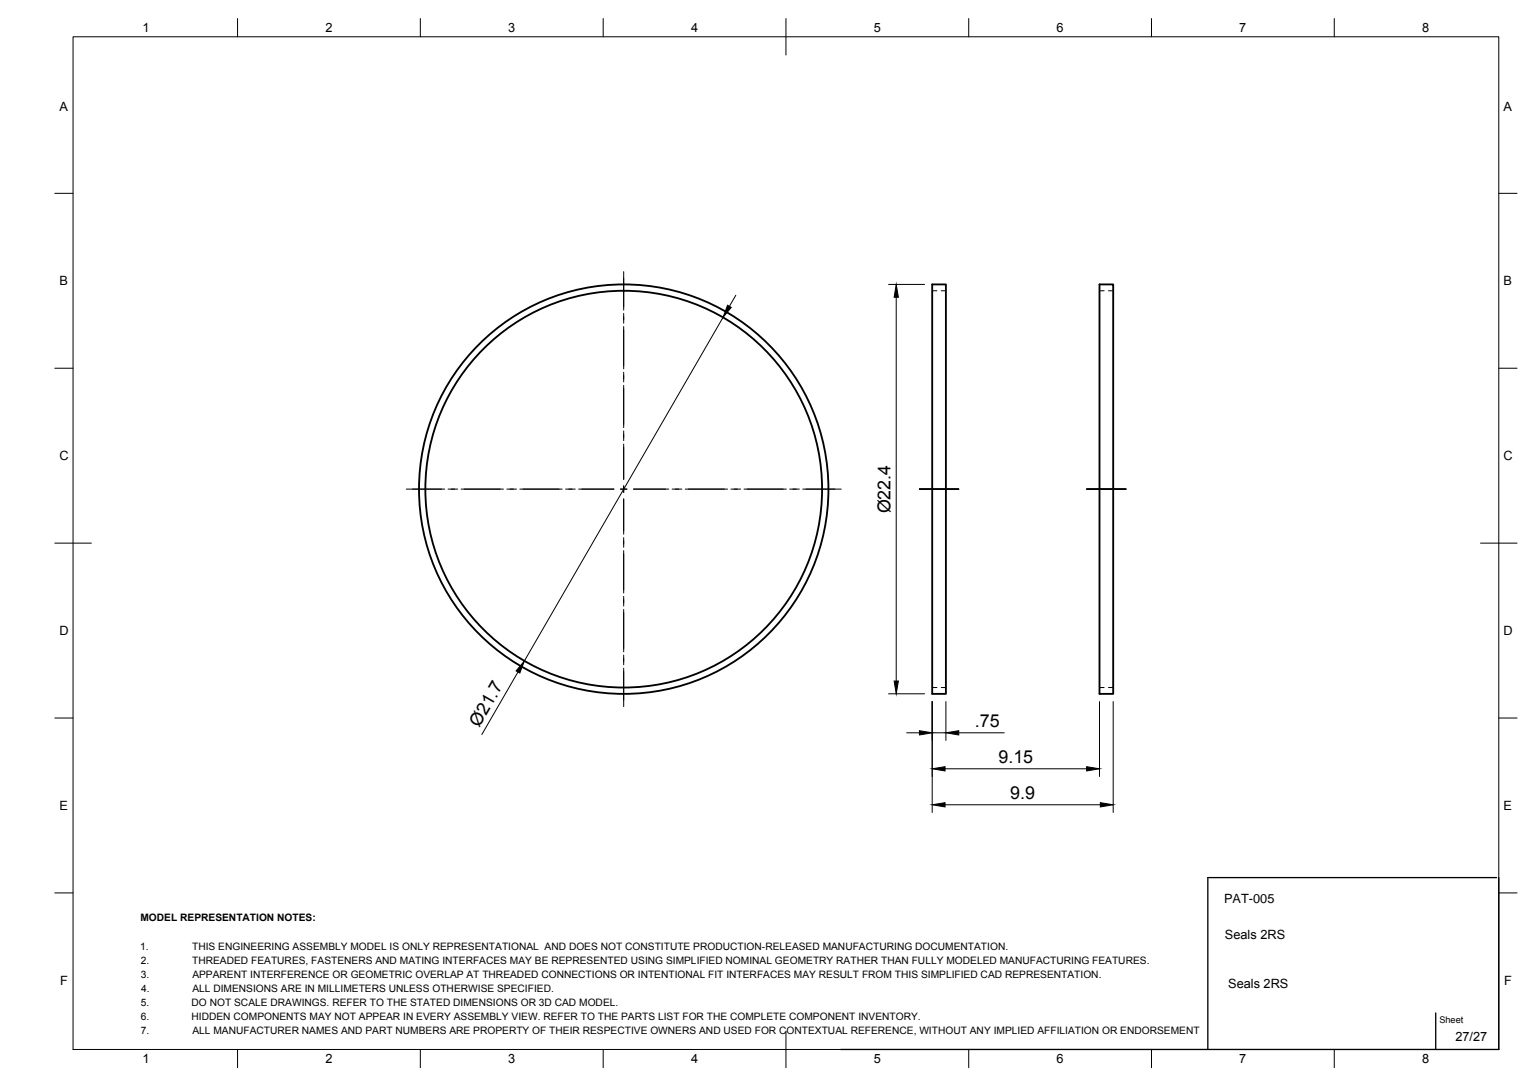
ISO-10303-21;
HEADER;
/* Generated by software containing ST-Developer
 * from STEP Tools, Inc. (www.steptools.com) 
 */

FILE_DESCRIPTION(
/* description */ ('Ball-race swivel caster'),
/* implementation_level */ '2;1');

FILE_NAME(
/* name */ 'Seals 2RS.step',
/* time_stamp */ '2026-10-29T16:15:51-07:00',
/* author */ (''),
/* organization */ (''),
/* preprocessor_version */ 'ST-DEVELOPER v20.2',
/* originating_system */ 'Autodesk Translation Framework v15.17.0.0',
/* authorisation */ '');

FILE_SCHEMA (('AUTOMOTIVE_DESIGN { 1 0 10303 214 3 1 1 }'));
ENDSEC;

DATA;
#10=MECHANICAL_DESIGN_GEOMETRIC_PRESENTATION_REPRESENTATION('',(#331,#332),#7816);
#276=SHAPE_REPRESENTATION_RELATIONSHIP('SRR','None',#7925,#296);
#296=ADVANCED_BREP_SHAPE_REPRESENTATION('',(#366,#367),#7814);
#331=STYLED_ITEM('',(#8097),#366);
#332=STYLED_ITEM('',(#8097),#367);
#366=MANIFOLD_SOLID_BREP('Body1',#3738);
#367=MANIFOLD_SOLID_BREP('Body2',#3739);
#432=FACE_BOUND('',#994,.T.);
#433=FACE_BOUND('',#997,.T.);
#434=FACE_BOUND('',#1000,.T.);
#435=FACE_BOUND('',#1003,.T.);
#518=PLANE('',#4451);
#519=PLANE('',#4456);
#520=PLANE('',#4459);
#521=PLANE('',#4464);
#721=FACE_OUTER_BOUND('',#993,.T.);
#722=FACE_OUTER_BOUND('',#995,.T.);
#723=FACE_OUTER_BOUND('',#996,.T.);
#724=FACE_OUTER_BOUND('',#998,.T.);
#725=FACE_OUTER_BOUND('',#999,.T.);
#726=FACE_OUTER_BOUND('',#1001,.T.);
#727=FACE_OUTER_BOUND('',#1002,.T.);
#728=FACE_OUTER_BOUND('',#1004,.T.);
#993=EDGE_LOOP('',(#3391));
#994=EDGE_LOOP('',(#3392));
#995=EDGE_LOOP('',(#3393,#3394,#3395,#3396));
#996=EDGE_LOOP('',(#3397));
#997=EDGE_LOOP('',(#3398));
#998=EDGE_LOOP('',(#3399,#3400,#3401,#3402));
#999=EDGE_LOOP('',(#3403));
#1000=EDGE_LOOP('',(#3404));
#1001=EDGE_LOOP('',(#3405,#3406,#3407,#3408));
#1002=EDGE_LOOP('',(#3409));
#1003=EDGE_LOOP('',(#3410));
#1004=EDGE_LOOP('',(#3411,#3412,#3413,#3414));
#1160=LINE('',#7715,#1315);
#1161=LINE('',#7720,#1316);
#1162=LINE('',#7729,#1317);
#1163=LINE('',#7734,#1318);
#1315=VECTOR('',#5626,1.119765);
#1316=VECTOR('',#5633,1.085235);
#1317=VECTOR('',#5644,1.119765);
#1318=VECTOR('',#5651,1.085235);
#1573=CIRCLE('',#4452,1.119765);
#1574=CIRCLE('',#4453,1.085235);
#1575=CIRCLE('',#4455,1.119765);
#1576=CIRCLE('',#4457,1.085235);
#1577=CIRCLE('',#4460,1.119765);
#1578=CIRCLE('',#4461,1.085235);
#1579=CIRCLE('',#4463,1.119765);
#1580=CIRCLE('',#4465,1.085235);
#1924=VERTEX_POINT('',#7708);
#1925=VERTEX_POINT('',#7710);
#1926=VERTEX_POINT('',#7713);
#1927=VERTEX_POINT('',#7717);
#1928=VERTEX_POINT('',#7722);
#1929=VERTEX_POINT('',#7724);
#1930=VERTEX_POINT('',#7727);
#1931=VERTEX_POINT('',#7731);
#2415=EDGE_CURVE('',#1924,#1924,#1573,.T.);
#2416=EDGE_CURVE('',#1925,#1925,#1574,.T.);
#2417=EDGE_CURVE('',#1926,#1926,#1575,.T.);
#2418=EDGE_CURVE('',#1926,#1924,#1160,.T.);
#2419=EDGE_CURVE('',#1927,#1927,#1576,.T.);
#2420=EDGE_CURVE('',#1927,#1925,#1161,.T.);
#2421=EDGE_CURVE('',#1928,#1928,#1577,.T.);
#2422=EDGE_CURVE('',#1929,#1929,#1578,.T.);
#2423=EDGE_CURVE('',#1930,#1930,#1579,.T.);
#2424=EDGE_CURVE('',#1930,#1928,#1162,.T.);
#2425=EDGE_CURVE('',#1931,#1931,#1580,.T.);
#2426=EDGE_CURVE('',#1931,#1929,#1163,.T.);
#3391=ORIENTED_EDGE('',*,*,#2415,.F.);
#3392=ORIENTED_EDGE('',*,*,#2416,.T.);
#3393=ORIENTED_EDGE('',*,*,#2417,.F.);
#3394=ORIENTED_EDGE('',*,*,#2418,.T.);
#3395=ORIENTED_EDGE('',*,*,#2415,.T.);
#3396=ORIENTED_EDGE('',*,*,#2418,.F.);
#3397=ORIENTED_EDGE('',*,*,#2417,.T.);
#3398=ORIENTED_EDGE('',*,*,#2419,.F.);
#3399=ORIENTED_EDGE('',*,*,#2419,.T.);
#3400=ORIENTED_EDGE('',*,*,#2420,.T.);
#3401=ORIENTED_EDGE('',*,*,#2416,.F.);
#3402=ORIENTED_EDGE('',*,*,#2420,.F.);
#3403=ORIENTED_EDGE('',*,*,#2421,.F.);
#3404=ORIENTED_EDGE('',*,*,#2422,.T.);
#3405=ORIENTED_EDGE('',*,*,#2423,.F.);
#3406=ORIENTED_EDGE('',*,*,#2424,.T.);
#3407=ORIENTED_EDGE('',*,*,#2421,.T.);
#3408=ORIENTED_EDGE('',*,*,#2424,.F.);
#3409=ORIENTED_EDGE('',*,*,#2423,.T.);
#3410=ORIENTED_EDGE('',*,*,#2425,.F.);
#3411=ORIENTED_EDGE('',*,*,#2425,.T.);
#3412=ORIENTED_EDGE('',*,*,#2426,.T.);
#3413=ORIENTED_EDGE('',*,*,#2422,.F.);
#3414=ORIENTED_EDGE('',*,*,#2426,.F.);
#3489=CYLINDRICAL_SURFACE('',#4454,1.119765);
#3490=CYLINDRICAL_SURFACE('',#4458,1.085235);
#3491=CYLINDRICAL_SURFACE('',#4462,1.119765);
#3492=CYLINDRICAL_SURFACE('',#4466,1.085235);
#3692=ADVANCED_FACE('',(#721,#432),#518,.T.);
#3693=ADVANCED_FACE('',(#722),#3489,.T.);
#3694=ADVANCED_FACE('',(#723,#433),#519,.T.);
#3695=ADVANCED_FACE('',(#724),#3490,.F.);
#3696=ADVANCED_FACE('',(#725,#434),#520,.T.);
#3697=ADVANCED_FACE('',(#726),#3491,.T.);
#3698=ADVANCED_FACE('',(#727,#435),#521,.T.);
#3699=ADVANCED_FACE('',(#728),#3492,.F.);
#3738=CLOSED_SHELL('',(#3692,#3693,#3694,#3695));
#3739=CLOSED_SHELL('',(#3696,#3697,#3698,#3699));
#4450=AXIS2_PLACEMENT_3D('',#7706,#5614,#5615);
#4451=AXIS2_PLACEMENT_3D('',#7707,#5616,#5617);
#4452=AXIS2_PLACEMENT_3D('',#7709,#5618,#5619);
#4453=AXIS2_PLACEMENT_3D('',#7711,#5620,#5621);
#4454=AXIS2_PLACEMENT_3D('',#7712,#5622,#5623);
#4455=AXIS2_PLACEMENT_3D('',#7714,#5624,#5625);
#4456=AXIS2_PLACEMENT_3D('',#7716,#5627,#5628);
#4457=AXIS2_PLACEMENT_3D('',#7718,#5629,#5630);
#4458=AXIS2_PLACEMENT_3D('',#7719,#5631,#5632);
#4459=AXIS2_PLACEMENT_3D('',#7721,#5634,#5635);
#4460=AXIS2_PLACEMENT_3D('',#7723,#5636,#5637);
#4461=AXIS2_PLACEMENT_3D('',#7725,#5638,#5639);
#4462=AXIS2_PLACEMENT_3D('',#7726,#5640,#5641);
#4463=AXIS2_PLACEMENT_3D('',#7728,#5642,#5643);
#4464=AXIS2_PLACEMENT_3D('',#7730,#5645,#5646);
#4465=AXIS2_PLACEMENT_3D('',#7732,#5647,#5648);
#4466=AXIS2_PLACEMENT_3D('',#7733,#5649,#5650);
#5614=DIRECTION('axis',(0.,0.,1.));
#5615=DIRECTION('refdir',(1.,0.,0.));
#5616=DIRECTION('center_axis',(0.,1.,0.));
#5617=DIRECTION('ref_axis',(0.,0.,1.));
#5618=DIRECTION('center_axis',(0.,-1.,0.));
#5619=DIRECTION('ref_axis',(1.,0.,0.));
#5620=DIRECTION('center_axis',(0.,-1.,0.));
#5621=DIRECTION('ref_axis',(1.,0.,0.));
#5622=DIRECTION('center_axis',(0.,-1.,0.));
#5623=DIRECTION('ref_axis',(1.,0.,0.));
#5624=DIRECTION('center_axis',(0.,-1.,0.));
#5625=DIRECTION('ref_axis',(1.,0.,0.));
#5626=DIRECTION('',(0.,1.,0.));
#5627=DIRECTION('center_axis',(0.,-1.,0.));
#5628=DIRECTION('ref_axis',(0.,0.,-1.));
#5629=DIRECTION('center_axis',(0.,-1.,0.));
#5630=DIRECTION('ref_axis',(1.,0.,0.));
#5631=DIRECTION('center_axis',(0.,-1.,0.));
#5632=DIRECTION('ref_axis',(1.,0.,0.));
#5633=DIRECTION('',(0.,1.,0.));
#5634=DIRECTION('center_axis',(0.,1.,0.));
#5635=DIRECTION('ref_axis',(0.,0.,1.));
#5636=DIRECTION('center_axis',(0.,-1.,0.));
#5637=DIRECTION('ref_axis',(1.,0.,0.));
#5638=DIRECTION('center_axis',(0.,-1.,0.));
#5639=DIRECTION('ref_axis',(1.,0.,0.));
#5640=DIRECTION('center_axis',(0.,-1.,0.));
#5641=DIRECTION('ref_axis',(1.,0.,0.));
#5642=DIRECTION('center_axis',(0.,-1.,0.));
#5643=DIRECTION('ref_axis',(1.,0.,0.));
#5644=DIRECTION('',(0.,1.,0.));
#5645=DIRECTION('center_axis',(0.,-1.,0.));
#5646=DIRECTION('ref_axis',(0.,0.,-1.));
#5647=DIRECTION('center_axis',(0.,-1.,0.));
#5648=DIRECTION('ref_axis',(1.,0.,0.));
#5649=DIRECTION('center_axis',(0.,-1.,0.));
#5650=DIRECTION('ref_axis',(1.,0.,0.));
#5651=DIRECTION('',(0.,1.,0.));
#7706=CARTESIAN_POINT('',(0.,0.,0.));
#7707=CARTESIAN_POINT('Origin',(1.119765,0.495,0.));
#7708=CARTESIAN_POINT('',(-1.119765,0.495,-1.37131662304724E-16));
#7709=CARTESIAN_POINT('Origin',(0.,0.495,0.));
#7710=CARTESIAN_POINT('',(-1.085235,0.495,-1.32902956907268E-16));
#7711=CARTESIAN_POINT('Origin',(0.,0.495,0.));
#7712=CARTESIAN_POINT('Origin',(0.,0.4575,0.));
#7713=CARTESIAN_POINT('',(-1.119765,0.42,-1.37131662304724E-16));
#7714=CARTESIAN_POINT('Origin',(0.,0.42,0.));
#7715=CARTESIAN_POINT('',(-1.119765,0.4575,-1.37131662304724E-16));
#7716=CARTESIAN_POINT('Origin',(1.085235,0.42,0.));
#7717=CARTESIAN_POINT('',(-1.085235,0.42,-1.32902956907268E-16));
#7718=CARTESIAN_POINT('Origin',(0.,0.42,0.));
#7719=CARTESIAN_POINT('Origin',(0.,0.4575,0.));
#7720=CARTESIAN_POINT('',(-1.085235,0.4575,-1.32902956907268E-16));
#7721=CARTESIAN_POINT('Origin',(1.119765,-0.42,0.));
#7722=CARTESIAN_POINT('',(-1.119765,-0.42,-1.37131662304724E-16));
#7723=CARTESIAN_POINT('Origin',(0.,-0.42,0.));
#7724=CARTESIAN_POINT('',(-1.085235,-0.42,-1.32902956907268E-16));
#7725=CARTESIAN_POINT('Origin',(0.,-0.42,0.));
#7726=CARTESIAN_POINT('Origin',(0.,-0.4575,0.));
#7727=CARTESIAN_POINT('',(-1.119765,-0.495,-1.37131662304724E-16));
#7728=CARTESIAN_POINT('Origin',(0.,-0.495,0.));
#7729=CARTESIAN_POINT('',(-1.119765,-0.4575,-1.37131662304724E-16));
#7730=CARTESIAN_POINT('Origin',(1.085235,-0.495,0.));
#7731=CARTESIAN_POINT('',(-1.085235,-0.495,-1.32902956907268E-16));
#7732=CARTESIAN_POINT('Origin',(0.,-0.495,0.));
#7733=CARTESIAN_POINT('Origin',(0.,-0.4575,0.));
#7734=CARTESIAN_POINT('',(-1.085235,-0.4575,-1.32902956907268E-16));
#7787=UNCERTAINTY_MEASURE_WITH_UNIT(LENGTH_MEASURE(0.001),#7817,
'DISTANCE_ACCURACY_VALUE',
'Maximum model space distance between geometric entities at asserted c
onnectivities');
#7789=UNCERTAINTY_MEASURE_WITH_UNIT(LENGTH_MEASURE(0.001),#7817,
'DISTANCE_ACCURACY_VALUE',
'Maximum model space distance between geometric entities at asserted c
onnectivities');
#7814=(
GEOMETRIC_REPRESENTATION_CONTEXT(3)
GLOBAL_UNCERTAINTY_ASSIGNED_CONTEXT((#7787))
GLOBAL_UNIT_ASSIGNED_CONTEXT((#7817,#7819,#7820))
REPRESENTATION_CONTEXT('','3D')
);
#7816=(
GEOMETRIC_REPRESENTATION_CONTEXT(3)
GLOBAL_UNCERTAINTY_ASSIGNED_CONTEXT((#7789))
GLOBAL_UNIT_ASSIGNED_CONTEXT((#7817,#7819,#7820))
REPRESENTATION_CONTEXT('','3D')
);
#7817=(
LENGTH_UNIT()
NAMED_UNIT(*)
SI_UNIT(.CENTI.,.METRE.)
);
#7819=(
NAMED_UNIT(*)
PLANE_ANGLE_UNIT()
SI_UNIT($,.RADIAN.)
);
#7820=(
NAMED_UNIT(*)
SI_UNIT($,.STERADIAN.)
SOLID_ANGLE_UNIT()
);
#7845=SHAPE_DEFINITION_REPRESENTATION(#7886,#7925);
#7886=PRODUCT_DEFINITION_SHAPE('',$,#7952);
#7925=SHAPE_REPRESENTATION('',(#4450),#7814);
#7927=PRODUCT_DEFINITION_CONTEXT('part definition',#8007,'design');
#7952=PRODUCT_DEFINITION('Seals 2RS','Seals 2RS',#7978,#7927);
#7978=PRODUCT_DEFINITION_FORMATION('',$,#8033);
#8007=APPLICATION_CONTEXT(
'Core Data for Automotive Mechanical Design Process');
#8008=PRODUCT_CONTEXT('part definition',#8007,'mechanical');
#8033=PRODUCT('Seals 2RS','Seals 2RS','Seals 2RS',(#8008));
#8091=COLOUR_RGB('Grey',0.48,0.52,0.57);
#8092=FILL_AREA_STYLE_COLOUR('',#8091);
#8093=FILL_AREA_STYLE('',(#8092));
#8094=SURFACE_STYLE_FILL_AREA(#8093);
#8095=SURFACE_SIDE_STYLE('',(#8094));
#8096=SURFACE_STYLE_USAGE(.BOTH.,#8095);
#8097=PRESENTATION_STYLE_ASSIGNMENT((#8096));
ENDSEC;
END-ISO-10303-21;
